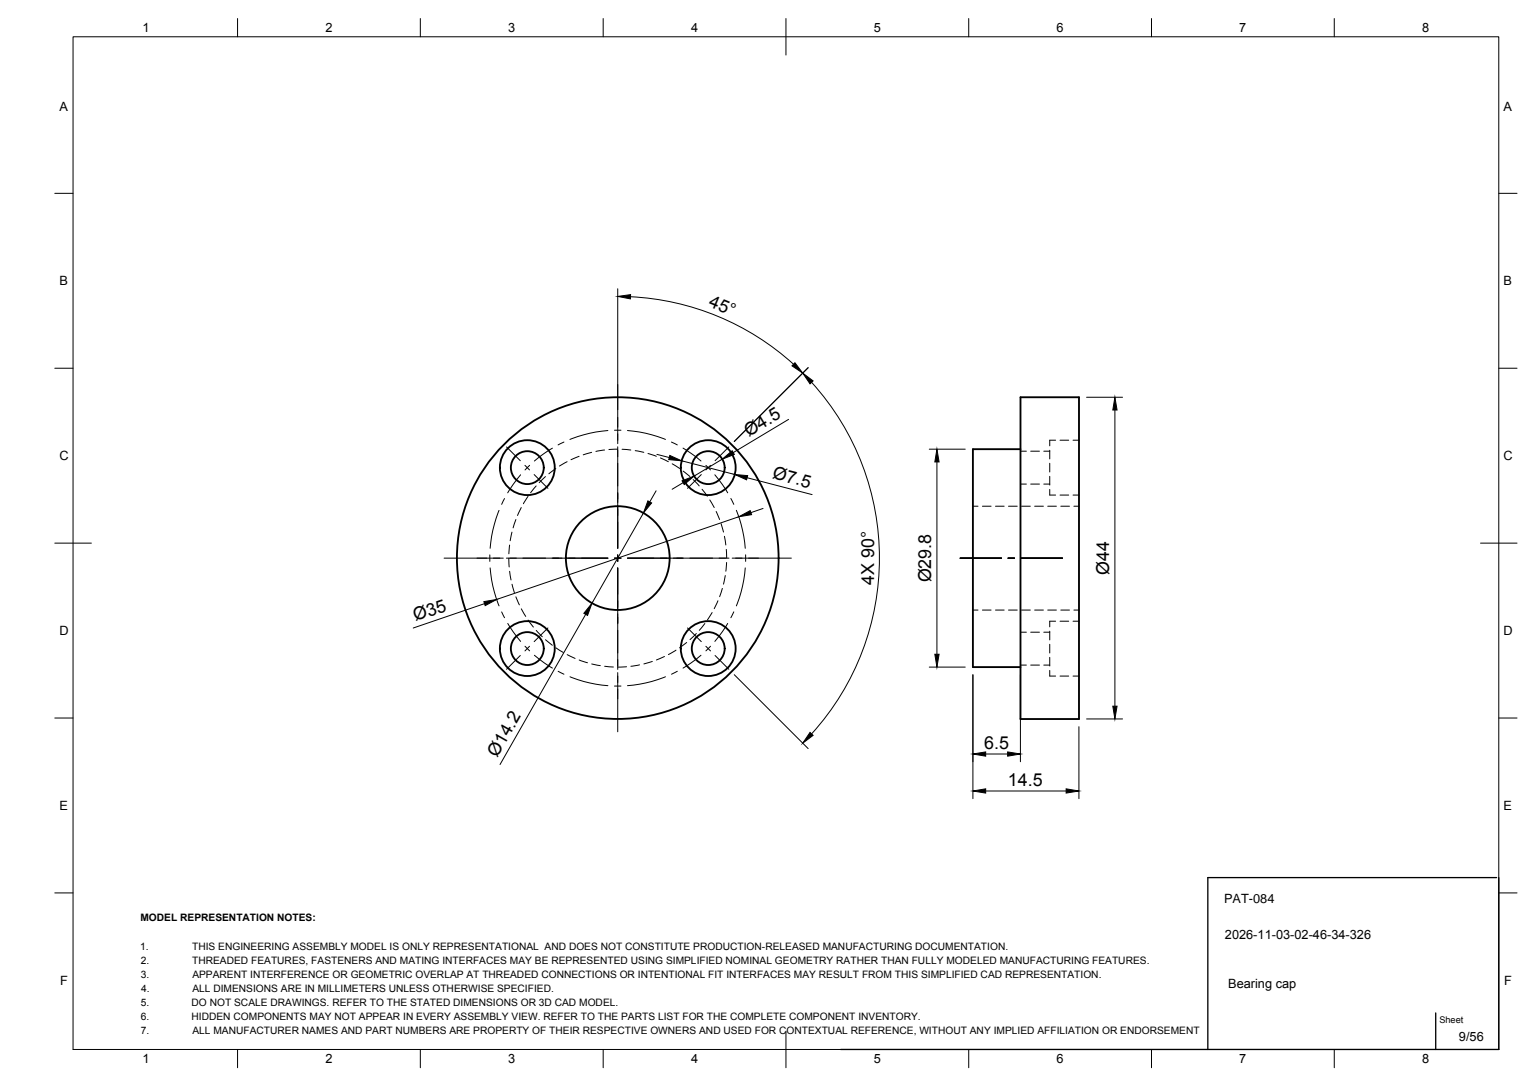
ISO-10303-21;
HEADER;
/* Generated by software containing ST-Developer
 * from STEP Tools, Inc. (www.steptools.com) 
 */

FILE_DESCRIPTION(
/* description */ ('Quick-return (Whitworth) mechanism'),
/* implementation_level */ '2;1');

FILE_NAME(
/* name */ 'Bearing cap.step',
/* time_stamp */ '2026-10-28T03:25:57-07:00',
/* author */ (''),
/* organization */ (''),
/* preprocessor_version */ 'ST-DEVELOPER v20.2',
/* originating_system */ 'Autodesk Translation Framework v15.17.0.0',
/* authorisation */ '');

FILE_SCHEMA (('AUTOMOTIVE_DESIGN { 1 0 10303 214 3 1 1 }'));
ENDSEC;

DATA;
#10=MECHANICAL_DESIGN_GEOMETRIC_PRESENTATION_REPRESENTATION('',(#494),#14878);
#406=SHAPE_REPRESENTATION_RELATIONSHIP('SRR','None',#15074,#450);
#450=ADVANCED_BREP_SHAPE_REPRESENTATION('',(#546),#14831);
#494=STYLED_ITEM('',(#15406),#546);
#546=MANIFOLD_SOLID_BREP('Body1',#7848);
#633=FACE_BOUND('',#1616,.T.);
#634=FACE_BOUND('',#1619,.T.);
#635=FACE_BOUND('',#1622,.T.);
#636=FACE_BOUND('',#1625,.T.);
#637=FACE_BOUND('',#1632,.T.);
#638=FACE_BOUND('',#1636,.T.);
#639=FACE_BOUND('',#1637,.T.);
#640=FACE_BOUND('',#1638,.T.);
#641=FACE_BOUND('',#1639,.T.);
#642=FACE_BOUND('',#1640,.T.);
#643=FACE_BOUND('',#1642,.T.);
#644=FACE_BOUND('',#1643,.T.);
#645=FACE_BOUND('',#1644,.T.);
#646=FACE_BOUND('',#1645,.T.);
#647=FACE_BOUND('',#1646,.T.);
#812=PLANE('',#8517);
#813=PLANE('',#8522);
#814=PLANE('',#8527);
#815=PLANE('',#8532);
#816=PLANE('',#8545);
#817=PLANE('',#8552);
#818=PLANE('',#8553);
#1106=FACE_OUTER_BOUND('',#1614,.T.);
#1107=FACE_OUTER_BOUND('',#1615,.T.);
#1108=FACE_OUTER_BOUND('',#1617,.T.);
#1109=FACE_OUTER_BOUND('',#1618,.T.);
#1110=FACE_OUTER_BOUND('',#1620,.T.);
#1111=FACE_OUTER_BOUND('',#1621,.T.);
#1112=FACE_OUTER_BOUND('',#1623,.T.);
#1113=FACE_OUTER_BOUND('',#1624,.T.);
#1114=FACE_OUTER_BOUND('',#1626,.T.);
#1115=FACE_OUTER_BOUND('',#1627,.T.);
#1116=FACE_OUTER_BOUND('',#1628,.T.);
#1117=FACE_OUTER_BOUND('',#1629,.T.);
#1118=FACE_OUTER_BOUND('',#1630,.T.);
#1119=FACE_OUTER_BOUND('',#1631,.T.);
#1120=FACE_OUTER_BOUND('',#1633,.T.);
#1121=FACE_OUTER_BOUND('',#1634,.T.);
#1122=FACE_OUTER_BOUND('',#1635,.T.);
#1123=FACE_OUTER_BOUND('',#1641,.T.);
#1614=EDGE_LOOP('',(#5536,#5537,#5538,#5539));
#1615=EDGE_LOOP('',(#5540));
#1616=EDGE_LOOP('',(#5541));
#1617=EDGE_LOOP('',(#5542,#5543,#5544,#5545));
#1618=EDGE_LOOP('',(#5546));
#1619=EDGE_LOOP('',(#5547));
#1620=EDGE_LOOP('',(#5548,#5549,#5550,#5551));
#1621=EDGE_LOOP('',(#5552));
#1622=EDGE_LOOP('',(#5553));
#1623=EDGE_LOOP('',(#5554,#5555,#5556,#5557));
#1624=EDGE_LOOP('',(#5558));
#1625=EDGE_LOOP('',(#5559));
#1626=EDGE_LOOP('',(#5560,#5561,#5562,#5563));
#1627=EDGE_LOOP('',(#5564,#5565,#5566,#5567));
#1628=EDGE_LOOP('',(#5568,#5569,#5570,#5571));
#1629=EDGE_LOOP('',(#5572,#5573,#5574,#5575));
#1630=EDGE_LOOP('',(#5576,#5577,#5578,#5579));
#1631=EDGE_LOOP('',(#5580));
#1632=EDGE_LOOP('',(#5581));
#1633=EDGE_LOOP('',(#5582,#5583,#5584,#5585));
#1634=EDGE_LOOP('',(#5586,#5587,#5588,#5589));
#1635=EDGE_LOOP('',(#5590));
#1636=EDGE_LOOP('',(#5591));
#1637=EDGE_LOOP('',(#5592));
#1638=EDGE_LOOP('',(#5593));
#1639=EDGE_LOOP('',(#5594));
#1640=EDGE_LOOP('',(#5595));
#1641=EDGE_LOOP('',(#5596));
#1642=EDGE_LOOP('',(#5597));
#1643=EDGE_LOOP('',(#5598));
#1644=EDGE_LOOP('',(#5599));
#1645=EDGE_LOOP('',(#5600));
#1646=EDGE_LOOP('',(#5601));
#2239=LINE('',#12313,#2762);
#2240=LINE('',#12322,#2763);
#2241=LINE('',#12331,#2764);
#2242=LINE('',#12340,#2765);
#2243=LINE('',#12348,#2766);
#2244=LINE('',#12352,#2767);
#2245=LINE('',#12356,#2768);
#2246=LINE('',#12360,#2769);
#2247=LINE('',#12365,#2770);
#2248=LINE('',#12373,#2771);
#2249=LINE('',#12378,#2772);
#2762=VECTOR('',#9730,0.375);
#2763=VECTOR('',#9741,0.375);
#2764=VECTOR('',#9752,0.375);
#2765=VECTOR('',#9763,0.375);
#2766=VECTOR('',#9774,0.225);
#2767=VECTOR('',#9779,0.225);
#2768=VECTOR('',#9784,0.225);
#2769=VECTOR('',#9789,0.225);
#2770=VECTOR('',#9794,1.49);
#2771=VECTOR('',#9805,0.71);
#2772=VECTOR('',#9810,2.2);
#3280=CIRCLE('',#8515,0.375);
#3281=CIRCLE('',#8516,0.375);
#3282=CIRCLE('',#8518,0.225);
#3283=CIRCLE('',#8520,0.375);
#3284=CIRCLE('',#8521,0.375);
#3285=CIRCLE('',#8523,0.225);
#3286=CIRCLE('',#8525,0.375);
#3287=CIRCLE('',#8526,0.375);
#3288=CIRCLE('',#8528,0.225);
#3289=CIRCLE('',#8530,0.375);
#3290=CIRCLE('',#8531,0.375);
#3291=CIRCLE('',#8533,0.225);
#3292=CIRCLE('',#8535,0.225);
#3293=CIRCLE('',#8537,0.225);
#3294=CIRCLE('',#8539,0.225);
#3295=CIRCLE('',#8541,0.225);
#3296=CIRCLE('',#8543,1.49);
#3297=CIRCLE('',#8544,1.49);
#3298=CIRCLE('',#8546,0.71);
#3299=CIRCLE('',#8548,0.71);
#3300=CIRCLE('',#8550,2.2);
#3301=CIRCLE('',#8551,2.2);
#3723=VERTEX_POINT('',#12310);
#3724=VERTEX_POINT('',#12312);
#3725=VERTEX_POINT('',#12316);
#3726=VERTEX_POINT('',#12319);
#3727=VERTEX_POINT('',#12321);
#3728=VERTEX_POINT('',#12325);
#3729=VERTEX_POINT('',#12328);
#3730=VERTEX_POINT('',#12330);
#3731=VERTEX_POINT('',#12334);
#3732=VERTEX_POINT('',#12337);
#3733=VERTEX_POINT('',#12339);
#3734=VERTEX_POINT('',#12343);
#3735=VERTEX_POINT('',#12346);
#3736=VERTEX_POINT('',#12350);
#3737=VERTEX_POINT('',#12354);
#3738=VERTEX_POINT('',#12358);
#3739=VERTEX_POINT('',#12362);
#3740=VERTEX_POINT('',#12364);
#3741=VERTEX_POINT('',#12368);
#3742=VERTEX_POINT('',#12371);
#3743=VERTEX_POINT('',#12375);
#3744=VERTEX_POINT('',#12377);
#4425=EDGE_CURVE('',#3723,#3723,#3280,.T.);
#4426=EDGE_CURVE('',#3723,#3724,#2239,.T.);
#4427=EDGE_CURVE('',#3724,#3724,#3281,.T.);
#4428=EDGE_CURVE('',#3725,#3725,#3282,.T.);
#4429=EDGE_CURVE('',#3726,#3726,#3283,.T.);
#4430=EDGE_CURVE('',#3726,#3727,#2240,.T.);
#4431=EDGE_CURVE('',#3727,#3727,#3284,.T.);
#4432=EDGE_CURVE('',#3728,#3728,#3285,.T.);
#4433=EDGE_CURVE('',#3729,#3729,#3286,.T.);
#4434=EDGE_CURVE('',#3729,#3730,#2241,.T.);
#4435=EDGE_CURVE('',#3730,#3730,#3287,.T.);
#4436=EDGE_CURVE('',#3731,#3731,#3288,.T.);
#4437=EDGE_CURVE('',#3732,#3732,#3289,.T.);
#4438=EDGE_CURVE('',#3732,#3733,#2242,.T.);
#4439=EDGE_CURVE('',#3733,#3733,#3290,.T.);
#4440=EDGE_CURVE('',#3734,#3734,#3291,.T.);
#4441=EDGE_CURVE('',#3735,#3735,#3292,.T.);
#4442=EDGE_CURVE('',#3735,#3725,#2243,.T.);
#4443=EDGE_CURVE('',#3736,#3736,#3293,.T.);
#4444=EDGE_CURVE('',#3736,#3728,#2244,.T.);
#4445=EDGE_CURVE('',#3737,#3737,#3294,.T.);
#4446=EDGE_CURVE('',#3737,#3731,#2245,.T.);
#4447=EDGE_CURVE('',#3738,#3738,#3295,.T.);
#4448=EDGE_CURVE('',#3738,#3734,#2246,.T.);
#4449=EDGE_CURVE('',#3739,#3739,#3296,.T.);
#4450=EDGE_CURVE('',#3739,#3740,#2247,.T.);
#4451=EDGE_CURVE('',#3740,#3740,#3297,.T.);
#4452=EDGE_CURVE('',#3741,#3741,#3298,.T.);
#4453=EDGE_CURVE('',#3742,#3742,#3299,.T.);
#4454=EDGE_CURVE('',#3742,#3741,#2248,.T.);
#4455=EDGE_CURVE('',#3743,#3743,#3300,.T.);
#4456=EDGE_CURVE('',#3743,#3744,#2249,.T.);
#4457=EDGE_CURVE('',#3744,#3744,#3301,.T.);
#5536=ORIENTED_EDGE('',*,*,#4425,.F.);
#5537=ORIENTED_EDGE('',*,*,#4426,.T.);
#5538=ORIENTED_EDGE('',*,*,#4427,.F.);
#5539=ORIENTED_EDGE('',*,*,#4426,.F.);
#5540=ORIENTED_EDGE('',*,*,#4425,.T.);
#5541=ORIENTED_EDGE('',*,*,#4428,.F.);
#5542=ORIENTED_EDGE('',*,*,#4429,.F.);
#5543=ORIENTED_EDGE('',*,*,#4430,.T.);
#5544=ORIENTED_EDGE('',*,*,#4431,.F.);
#5545=ORIENTED_EDGE('',*,*,#4430,.F.);
#5546=ORIENTED_EDGE('',*,*,#4429,.T.);
#5547=ORIENTED_EDGE('',*,*,#4432,.F.);
#5548=ORIENTED_EDGE('',*,*,#4433,.F.);
#5549=ORIENTED_EDGE('',*,*,#4434,.T.);
#5550=ORIENTED_EDGE('',*,*,#4435,.F.);
#5551=ORIENTED_EDGE('',*,*,#4434,.F.);
#5552=ORIENTED_EDGE('',*,*,#4433,.T.);
#5553=ORIENTED_EDGE('',*,*,#4436,.F.);
#5554=ORIENTED_EDGE('',*,*,#4437,.F.);
#5555=ORIENTED_EDGE('',*,*,#4438,.T.);
#5556=ORIENTED_EDGE('',*,*,#4439,.F.);
#5557=ORIENTED_EDGE('',*,*,#4438,.F.);
#5558=ORIENTED_EDGE('',*,*,#4437,.T.);
#5559=ORIENTED_EDGE('',*,*,#4440,.F.);
#5560=ORIENTED_EDGE('',*,*,#4441,.F.);
#5561=ORIENTED_EDGE('',*,*,#4442,.T.);
#5562=ORIENTED_EDGE('',*,*,#4428,.T.);
#5563=ORIENTED_EDGE('',*,*,#4442,.F.);
#5564=ORIENTED_EDGE('',*,*,#4443,.F.);
#5565=ORIENTED_EDGE('',*,*,#4444,.T.);
#5566=ORIENTED_EDGE('',*,*,#4432,.T.);
#5567=ORIENTED_EDGE('',*,*,#4444,.F.);
#5568=ORIENTED_EDGE('',*,*,#4445,.F.);
#5569=ORIENTED_EDGE('',*,*,#4446,.T.);
#5570=ORIENTED_EDGE('',*,*,#4436,.T.);
#5571=ORIENTED_EDGE('',*,*,#4446,.F.);
#5572=ORIENTED_EDGE('',*,*,#4447,.F.);
#5573=ORIENTED_EDGE('',*,*,#4448,.T.);
#5574=ORIENTED_EDGE('',*,*,#4440,.T.);
#5575=ORIENTED_EDGE('',*,*,#4448,.F.);
#5576=ORIENTED_EDGE('',*,*,#4449,.F.);
#5577=ORIENTED_EDGE('',*,*,#4450,.T.);
#5578=ORIENTED_EDGE('',*,*,#4451,.T.);
#5579=ORIENTED_EDGE('',*,*,#4450,.F.);
#5580=ORIENTED_EDGE('',*,*,#4451,.F.);
#5581=ORIENTED_EDGE('',*,*,#4452,.F.);
#5582=ORIENTED_EDGE('',*,*,#4453,.F.);
#5583=ORIENTED_EDGE('',*,*,#4454,.T.);
#5584=ORIENTED_EDGE('',*,*,#4452,.T.);
#5585=ORIENTED_EDGE('',*,*,#4454,.F.);
#5586=ORIENTED_EDGE('',*,*,#4455,.F.);
#5587=ORIENTED_EDGE('',*,*,#4456,.T.);
#5588=ORIENTED_EDGE('',*,*,#4457,.T.);
#5589=ORIENTED_EDGE('',*,*,#4456,.F.);
#5590=ORIENTED_EDGE('',*,*,#4455,.T.);
#5591=ORIENTED_EDGE('',*,*,#4453,.T.);
#5592=ORIENTED_EDGE('',*,*,#4439,.T.);
#5593=ORIENTED_EDGE('',*,*,#4435,.T.);
#5594=ORIENTED_EDGE('',*,*,#4431,.T.);
#5595=ORIENTED_EDGE('',*,*,#4427,.T.);
#5596=ORIENTED_EDGE('',*,*,#4457,.F.);
#5597=ORIENTED_EDGE('',*,*,#4449,.T.);
#5598=ORIENTED_EDGE('',*,*,#4447,.T.);
#5599=ORIENTED_EDGE('',*,*,#4445,.T.);
#5600=ORIENTED_EDGE('',*,*,#4443,.T.);
#5601=ORIENTED_EDGE('',*,*,#4441,.T.);
#7239=CYLINDRICAL_SURFACE('',#8514,0.375);
#7240=CYLINDRICAL_SURFACE('',#8519,0.375);
#7241=CYLINDRICAL_SURFACE('',#8524,0.375);
#7242=CYLINDRICAL_SURFACE('',#8529,0.375);
#7243=CYLINDRICAL_SURFACE('',#8534,0.225);
#7244=CYLINDRICAL_SURFACE('',#8536,0.225);
#7245=CYLINDRICAL_SURFACE('',#8538,0.225);
#7246=CYLINDRICAL_SURFACE('',#8540,0.225);
#7247=CYLINDRICAL_SURFACE('',#8542,1.49);
#7248=CYLINDRICAL_SURFACE('',#8547,0.71);
#7249=CYLINDRICAL_SURFACE('',#8549,2.2);
#7437=ADVANCED_FACE('',(#1106),#7239,.F.);
#7438=ADVANCED_FACE('',(#1107,#633),#812,.T.);
#7439=ADVANCED_FACE('',(#1108),#7240,.F.);
#7440=ADVANCED_FACE('',(#1109,#634),#813,.T.);
#7441=ADVANCED_FACE('',(#1110),#7241,.F.);
#7442=ADVANCED_FACE('',(#1111,#635),#814,.T.);
#7443=ADVANCED_FACE('',(#1112),#7242,.F.);
#7444=ADVANCED_FACE('',(#1113,#636),#815,.T.);
#7445=ADVANCED_FACE('',(#1114),#7243,.F.);
#7446=ADVANCED_FACE('',(#1115),#7244,.F.);
#7447=ADVANCED_FACE('',(#1116),#7245,.F.);
#7448=ADVANCED_FACE('',(#1117),#7246,.F.);
#7449=ADVANCED_FACE('',(#1118),#7247,.T.);
#7450=ADVANCED_FACE('',(#1119,#637),#816,.F.);
#7451=ADVANCED_FACE('',(#1120),#7248,.F.);
#7452=ADVANCED_FACE('',(#1121),#7249,.T.);
#7453=ADVANCED_FACE('',(#1122,#638,#639,#640,#641,#642),#817,.T.);
#7454=ADVANCED_FACE('',(#1123,#643,#644,#645,#646,#647),#818,.F.);
#7848=CLOSED_SHELL('',(#7437,#7438,#7439,#7440,#7441,#7442,#7443,#7444,
#7445,#7446,#7447,#7448,#7449,#7450,#7451,#7452,#7453,#7454));
#8513=AXIS2_PLACEMENT_3D('',#12308,#9724,#9725);
#8514=AXIS2_PLACEMENT_3D('',#12309,#9726,#9727);
#8515=AXIS2_PLACEMENT_3D('',#12311,#9728,#9729);
#8516=AXIS2_PLACEMENT_3D('',#12314,#9731,#9732);
#8517=AXIS2_PLACEMENT_3D('',#12315,#9733,#9734);
#8518=AXIS2_PLACEMENT_3D('',#12317,#9735,#9736);
#8519=AXIS2_PLACEMENT_3D('',#12318,#9737,#9738);
#8520=AXIS2_PLACEMENT_3D('',#12320,#9739,#9740);
#8521=AXIS2_PLACEMENT_3D('',#12323,#9742,#9743);
#8522=AXIS2_PLACEMENT_3D('',#12324,#9744,#9745);
#8523=AXIS2_PLACEMENT_3D('',#12326,#9746,#9747);
#8524=AXIS2_PLACEMENT_3D('',#12327,#9748,#9749);
#8525=AXIS2_PLACEMENT_3D('',#12329,#9750,#9751);
#8526=AXIS2_PLACEMENT_3D('',#12332,#9753,#9754);
#8527=AXIS2_PLACEMENT_3D('',#12333,#9755,#9756);
#8528=AXIS2_PLACEMENT_3D('',#12335,#9757,#9758);
#8529=AXIS2_PLACEMENT_3D('',#12336,#9759,#9760);
#8530=AXIS2_PLACEMENT_3D('',#12338,#9761,#9762);
#8531=AXIS2_PLACEMENT_3D('',#12341,#9764,#9765);
#8532=AXIS2_PLACEMENT_3D('',#12342,#9766,#9767);
#8533=AXIS2_PLACEMENT_3D('',#12344,#9768,#9769);
#8534=AXIS2_PLACEMENT_3D('',#12345,#9770,#9771);
#8535=AXIS2_PLACEMENT_3D('',#12347,#9772,#9773);
#8536=AXIS2_PLACEMENT_3D('',#12349,#9775,#9776);
#8537=AXIS2_PLACEMENT_3D('',#12351,#9777,#9778);
#8538=AXIS2_PLACEMENT_3D('',#12353,#9780,#9781);
#8539=AXIS2_PLACEMENT_3D('',#12355,#9782,#9783);
#8540=AXIS2_PLACEMENT_3D('',#12357,#9785,#9786);
#8541=AXIS2_PLACEMENT_3D('',#12359,#9787,#9788);
#8542=AXIS2_PLACEMENT_3D('',#12361,#9790,#9791);
#8543=AXIS2_PLACEMENT_3D('',#12363,#9792,#9793);
#8544=AXIS2_PLACEMENT_3D('',#12366,#9795,#9796);
#8545=AXIS2_PLACEMENT_3D('',#12367,#9797,#9798);
#8546=AXIS2_PLACEMENT_3D('',#12369,#9799,#9800);
#8547=AXIS2_PLACEMENT_3D('',#12370,#9801,#9802);
#8548=AXIS2_PLACEMENT_3D('',#12372,#9803,#9804);
#8549=AXIS2_PLACEMENT_3D('',#12374,#9806,#9807);
#8550=AXIS2_PLACEMENT_3D('',#12376,#9808,#9809);
#8551=AXIS2_PLACEMENT_3D('',#12379,#9811,#9812);
#8552=AXIS2_PLACEMENT_3D('',#12380,#9813,#9814);
#8553=AXIS2_PLACEMENT_3D('',#12381,#9815,#9816);
#9724=DIRECTION('axis',(0.,0.,1.));
#9725=DIRECTION('refdir',(1.,0.,0.));
#9726=DIRECTION('center_axis',(0.,0.,1.));
#9727=DIRECTION('ref_axis',(1.,0.,0.));
#9728=DIRECTION('center_axis',(0.,0.,1.));
#9729=DIRECTION('ref_axis',(1.,0.,0.));
#9730=DIRECTION('',(0.,0.,1.));
#9731=DIRECTION('center_axis',(0.,0.,-1.));
#9732=DIRECTION('ref_axis',(1.,0.,0.));
#9733=DIRECTION('center_axis',(0.,0.,1.));
#9734=DIRECTION('ref_axis',(1.,0.,0.));
#9735=DIRECTION('center_axis',(0.,0.,1.));
#9736=DIRECTION('ref_axis',(1.,0.,0.));
#9737=DIRECTION('center_axis',(0.,0.,1.));
#9738=DIRECTION('ref_axis',(1.,0.,0.));
#9739=DIRECTION('center_axis',(0.,0.,1.));
#9740=DIRECTION('ref_axis',(1.,0.,0.));
#9741=DIRECTION('',(0.,0.,1.));
#9742=DIRECTION('center_axis',(0.,0.,-1.));
#9743=DIRECTION('ref_axis',(1.,0.,0.));
#9744=DIRECTION('center_axis',(0.,0.,1.));
#9745=DIRECTION('ref_axis',(1.,0.,0.));
#9746=DIRECTION('center_axis',(0.,0.,1.));
#9747=DIRECTION('ref_axis',(1.,0.,0.));
#9748=DIRECTION('center_axis',(0.,0.,1.));
#9749=DIRECTION('ref_axis',(1.,0.,0.));
#9750=DIRECTION('center_axis',(0.,0.,1.));
#9751=DIRECTION('ref_axis',(1.,0.,0.));
#9752=DIRECTION('',(0.,0.,1.));
#9753=DIRECTION('center_axis',(0.,0.,-1.));
#9754=DIRECTION('ref_axis',(1.,0.,0.));
#9755=DIRECTION('center_axis',(0.,0.,1.));
#9756=DIRECTION('ref_axis',(1.,0.,0.));
#9757=DIRECTION('center_axis',(0.,0.,1.));
#9758=DIRECTION('ref_axis',(1.,0.,0.));
#9759=DIRECTION('center_axis',(0.,0.,1.));
#9760=DIRECTION('ref_axis',(1.,0.,0.));
#9761=DIRECTION('center_axis',(0.,0.,1.));
#9762=DIRECTION('ref_axis',(1.,0.,0.));
#9763=DIRECTION('',(0.,0.,1.));
#9764=DIRECTION('center_axis',(0.,0.,-1.));
#9765=DIRECTION('ref_axis',(1.,0.,0.));
#9766=DIRECTION('center_axis',(0.,0.,1.));
#9767=DIRECTION('ref_axis',(1.,0.,0.));
#9768=DIRECTION('center_axis',(0.,0.,1.));
#9769=DIRECTION('ref_axis',(1.,0.,0.));
#9770=DIRECTION('center_axis',(0.,0.,1.));
#9771=DIRECTION('ref_axis',(1.,0.,0.));
#9772=DIRECTION('center_axis',(0.,0.,1.));
#9773=DIRECTION('ref_axis',(1.,0.,0.));
#9774=DIRECTION('',(0.,0.,1.));
#9775=DIRECTION('center_axis',(0.,0.,1.));
#9776=DIRECTION('ref_axis',(1.,0.,0.));
#9777=DIRECTION('center_axis',(0.,0.,1.));
#9778=DIRECTION('ref_axis',(1.,0.,0.));
#9779=DIRECTION('',(0.,0.,1.));
#9780=DIRECTION('center_axis',(0.,0.,1.));
#9781=DIRECTION('ref_axis',(1.,0.,0.));
#9782=DIRECTION('center_axis',(0.,0.,1.));
#9783=DIRECTION('ref_axis',(1.,0.,0.));
#9784=DIRECTION('',(0.,0.,1.));
#9785=DIRECTION('center_axis',(0.,0.,1.));
#9786=DIRECTION('ref_axis',(1.,0.,0.));
#9787=DIRECTION('center_axis',(0.,0.,1.));
#9788=DIRECTION('ref_axis',(1.,0.,0.));
#9789=DIRECTION('',(0.,0.,1.));
#9790=DIRECTION('center_axis',(0.,0.,1.));
#9791=DIRECTION('ref_axis',(1.,0.,0.));
#9792=DIRECTION('center_axis',(0.,0.,1.));
#9793=DIRECTION('ref_axis',(1.,0.,0.));
#9794=DIRECTION('',(0.,0.,-1.));
#9795=DIRECTION('center_axis',(0.,0.,1.));
#9796=DIRECTION('ref_axis',(1.,0.,0.));
#9797=DIRECTION('center_axis',(0.,0.,1.));
#9798=DIRECTION('ref_axis',(1.,0.,0.));
#9799=DIRECTION('center_axis',(0.,0.,-1.));
#9800=DIRECTION('ref_axis',(1.,0.,0.));
#9801=DIRECTION('center_axis',(0.,0.,1.));
#9802=DIRECTION('ref_axis',(1.,0.,0.));
#9803=DIRECTION('center_axis',(0.,0.,-1.));
#9804=DIRECTION('ref_axis',(1.,0.,0.));
#9805=DIRECTION('',(0.,0.,-1.));
#9806=DIRECTION('center_axis',(0.,0.,1.));
#9807=DIRECTION('ref_axis',(1.,0.,0.));
#9808=DIRECTION('center_axis',(0.,0.,1.));
#9809=DIRECTION('ref_axis',(1.,0.,0.));
#9810=DIRECTION('',(0.,0.,-1.));
#9811=DIRECTION('center_axis',(0.,0.,1.));
#9812=DIRECTION('ref_axis',(1.,0.,0.));
#9813=DIRECTION('center_axis',(0.,0.,1.));
#9814=DIRECTION('ref_axis',(1.,0.,0.));
#9815=DIRECTION('center_axis',(0.,0.,1.));
#9816=DIRECTION('ref_axis',(1.,0.,0.));
#12308=CARTESIAN_POINT('',(0.,0.,0.));
#12309=CARTESIAN_POINT('Origin',(-1.23743686707646,-1.23743686707646,4.));
#12310=CARTESIAN_POINT('',(-1.61243686707646,-1.23743686707646,4.));
#12311=CARTESIAN_POINT('Origin',(-1.23743686707646,-1.23743686707646,4.));
#12312=CARTESIAN_POINT('',(-1.61243686707646,-1.23743686707646,4.4));
#12313=CARTESIAN_POINT('',(-1.61243686707646,-1.23743686707646,4.));
#12314=CARTESIAN_POINT('Origin',(-1.23743686707646,-1.23743686707646,4.4));
#12315=CARTESIAN_POINT('Origin',(-1.23743686707646,-1.23743686707646,4.));
#12316=CARTESIAN_POINT('',(-1.46243686707646,-1.23743686707646,4.));
#12317=CARTESIAN_POINT('Origin',(-1.23743686707646,-1.23743686707646,4.));
#12318=CARTESIAN_POINT('Origin',(-1.23743686707646,1.23743686707646,4.));
#12319=CARTESIAN_POINT('',(-1.61243686707646,1.23743686707646,4.));
#12320=CARTESIAN_POINT('Origin',(-1.23743686707646,1.23743686707646,4.));
#12321=CARTESIAN_POINT('',(-1.61243686707646,1.23743686707646,4.4));
#12322=CARTESIAN_POINT('',(-1.61243686707646,1.23743686707646,4.));
#12323=CARTESIAN_POINT('Origin',(-1.23743686707646,1.23743686707646,4.4));
#12324=CARTESIAN_POINT('Origin',(-1.23743686707646,1.23743686707646,4.));
#12325=CARTESIAN_POINT('',(-1.46243686707646,1.23743686707646,4.));
#12326=CARTESIAN_POINT('Origin',(-1.23743686707646,1.23743686707646,4.));
#12327=CARTESIAN_POINT('Origin',(1.23743686707646,1.23743686707646,4.));
#12328=CARTESIAN_POINT('',(0.862436867076458,1.23743686707646,4.));
#12329=CARTESIAN_POINT('Origin',(1.23743686707646,1.23743686707646,4.));
#12330=CARTESIAN_POINT('',(0.862436867076458,1.23743686707646,4.4));
#12331=CARTESIAN_POINT('',(0.862436867076458,1.23743686707646,4.));
#12332=CARTESIAN_POINT('Origin',(1.23743686707646,1.23743686707646,4.4));
#12333=CARTESIAN_POINT('Origin',(1.23743686707646,1.23743686707646,4.));
#12334=CARTESIAN_POINT('',(1.01243686707646,1.23743686707646,4.));
#12335=CARTESIAN_POINT('Origin',(1.23743686707646,1.23743686707646,4.));
#12336=CARTESIAN_POINT('Origin',(1.23743686707646,-1.23743686707646,4.));
#12337=CARTESIAN_POINT('',(0.862436867076458,-1.23743686707646,4.));
#12338=CARTESIAN_POINT('Origin',(1.23743686707646,-1.23743686707646,4.));
#12339=CARTESIAN_POINT('',(0.862436867076458,-1.23743686707646,4.4));
#12340=CARTESIAN_POINT('',(0.862436867076458,-1.23743686707646,4.));
#12341=CARTESIAN_POINT('Origin',(1.23743686707646,-1.23743686707646,4.4));
#12342=CARTESIAN_POINT('Origin',(1.23743686707646,-1.23743686707646,4.));
#12343=CARTESIAN_POINT('',(1.01243686707646,-1.23743686707646,4.));
#12344=CARTESIAN_POINT('Origin',(1.23743686707646,-1.23743686707646,4.));
#12345=CARTESIAN_POINT('Origin',(-1.23743686707646,-1.23743686707646,3.5));
#12346=CARTESIAN_POINT('',(-1.46243686707646,-1.23743686707646,3.6));
#12347=CARTESIAN_POINT('Origin',(-1.23743686707646,-1.23743686707646,3.6));
#12348=CARTESIAN_POINT('',(-1.46243686707646,-1.23743686707646,3.5));
#12349=CARTESIAN_POINT('Origin',(-1.23743686707646,1.23743686707646,3.5));
#12350=CARTESIAN_POINT('',(-1.46243686707646,1.23743686707646,3.6));
#12351=CARTESIAN_POINT('Origin',(-1.23743686707646,1.23743686707646,3.6));
#12352=CARTESIAN_POINT('',(-1.46243686707646,1.23743686707646,3.5));
#12353=CARTESIAN_POINT('Origin',(1.23743686707646,1.23743686707646,3.5));
#12354=CARTESIAN_POINT('',(1.01243686707646,1.23743686707646,3.6));
#12355=CARTESIAN_POINT('Origin',(1.23743686707646,1.23743686707646,3.6));
#12356=CARTESIAN_POINT('',(1.01243686707646,1.23743686707646,3.5));
#12357=CARTESIAN_POINT('Origin',(1.23743686707646,-1.23743686707646,3.5));
#12358=CARTESIAN_POINT('',(1.01243686707646,-1.23743686707646,3.6));
#12359=CARTESIAN_POINT('Origin',(1.23743686707646,-1.23743686707646,3.6));
#12360=CARTESIAN_POINT('',(1.01243686707646,-1.23743686707646,3.5));
#12361=CARTESIAN_POINT('Origin',(0.,0.,2.95));
#12362=CARTESIAN_POINT('',(-1.49,-1.82472373072956E-16,3.6));
#12363=CARTESIAN_POINT('Origin',(0.,0.,3.6));
#12364=CARTESIAN_POINT('',(-1.49,-1.82472373072956E-16,2.95));
#12365=CARTESIAN_POINT('',(-1.49,-1.82472373072956E-16,2.95));
#12366=CARTESIAN_POINT('Origin',(0.,0.,2.95));
#12367=CARTESIAN_POINT('Origin',(0.,0.,2.95));
#12368=CARTESIAN_POINT('',(-0.71,-8.69499227394621E-17,2.95));
#12369=CARTESIAN_POINT('Origin',(0.,0.,2.95));
#12370=CARTESIAN_POINT('Origin',(0.,0.,3.6));
#12371=CARTESIAN_POINT('',(-0.71,-8.69499227394621E-17,4.4));
#12372=CARTESIAN_POINT('Origin',(0.,0.,4.4));
#12373=CARTESIAN_POINT('',(-0.71,-8.69499227394621E-17,3.6));
#12374=CARTESIAN_POINT('Origin',(0.,0.,3.6));
#12375=CARTESIAN_POINT('',(-2.2,-2.69422295812418E-16,4.4));
#12376=CARTESIAN_POINT('Origin',(0.,0.,4.4));
#12377=CARTESIAN_POINT('',(-2.2,-2.69422295812418E-16,3.6));
#12378=CARTESIAN_POINT('',(-2.2,-2.69422295812418E-16,3.6));
#12379=CARTESIAN_POINT('Origin',(0.,0.,3.6));
#12380=CARTESIAN_POINT('Origin',(0.,0.,4.4));
#12381=CARTESIAN_POINT('Origin',(0.,0.,3.6));
#14777=UNCERTAINTY_MEASURE_WITH_UNIT(LENGTH_MEASURE(0.001),#14879,
'DISTANCE_ACCURACY_VALUE',
'Maximum model space distance between geometric entities at asserted c
onnectivities');
#14824=UNCERTAINTY_MEASURE_WITH_UNIT(LENGTH_MEASURE(0.001),#14879,
'DISTANCE_ACCURACY_VALUE',
'Maximum model space distance between geometric entities at asserted c
onnectivities');
#14831=(
GEOMETRIC_REPRESENTATION_CONTEXT(3)
GLOBAL_UNCERTAINTY_ASSIGNED_CONTEXT((#14777))
GLOBAL_UNIT_ASSIGNED_CONTEXT((#14879,#14881,#14882))
REPRESENTATION_CONTEXT('','3D')
);
#14878=(
GEOMETRIC_REPRESENTATION_CONTEXT(3)
GLOBAL_UNCERTAINTY_ASSIGNED_CONTEXT((#14824))
GLOBAL_UNIT_ASSIGNED_CONTEXT((#14879,#14881,#14882))
REPRESENTATION_CONTEXT('','3D')
);
#14879=(
LENGTH_UNIT()
NAMED_UNIT(*)
SI_UNIT(.CENTI.,.METRE.)
);
#14881=(
NAMED_UNIT(*)
PLANE_ANGLE_UNIT()
SI_UNIT($,.RADIAN.)
);
#14882=(
NAMED_UNIT(*)
SI_UNIT($,.STERADIAN.)
SOLID_ANGLE_UNIT()
);
#14889=SHAPE_DEFINITION_REPRESENTATION(#14942,#15074);
#14942=PRODUCT_DEFINITION_SHAPE('',$,#15128);
#15074=SHAPE_REPRESENTATION('',(#8513),#14831);
#15121=PRODUCT_DEFINITION_CONTEXT('part definition',#15282,'design');
#15128=PRODUCT_DEFINITION('Bearing cap','Bearing cap',#15181,#15121);
#15181=PRODUCT_DEFINITION_FORMATION('',$,#15290);
#15282=APPLICATION_CONTEXT(
'Core Data for Automotive Mechanical Design Process');
#15283=PRODUCT_CONTEXT('part definition',#15282,'mechanical');
#15290=PRODUCT('Bearing cap','Bearing cap','Bearing cap',(#15283));
#15400=COLOUR_RGB('Grey',0.48,0.52,0.57);
#15401=FILL_AREA_STYLE_COLOUR('',#15400);
#15402=FILL_AREA_STYLE('',(#15401));
#15403=SURFACE_STYLE_FILL_AREA(#15402);
#15404=SURFACE_SIDE_STYLE('',(#15403));
#15405=SURFACE_STYLE_USAGE(.BOTH.,#15404);
#15406=PRESENTATION_STYLE_ASSIGNMENT((#15405));
ENDSEC;
END-ISO-10303-21;
